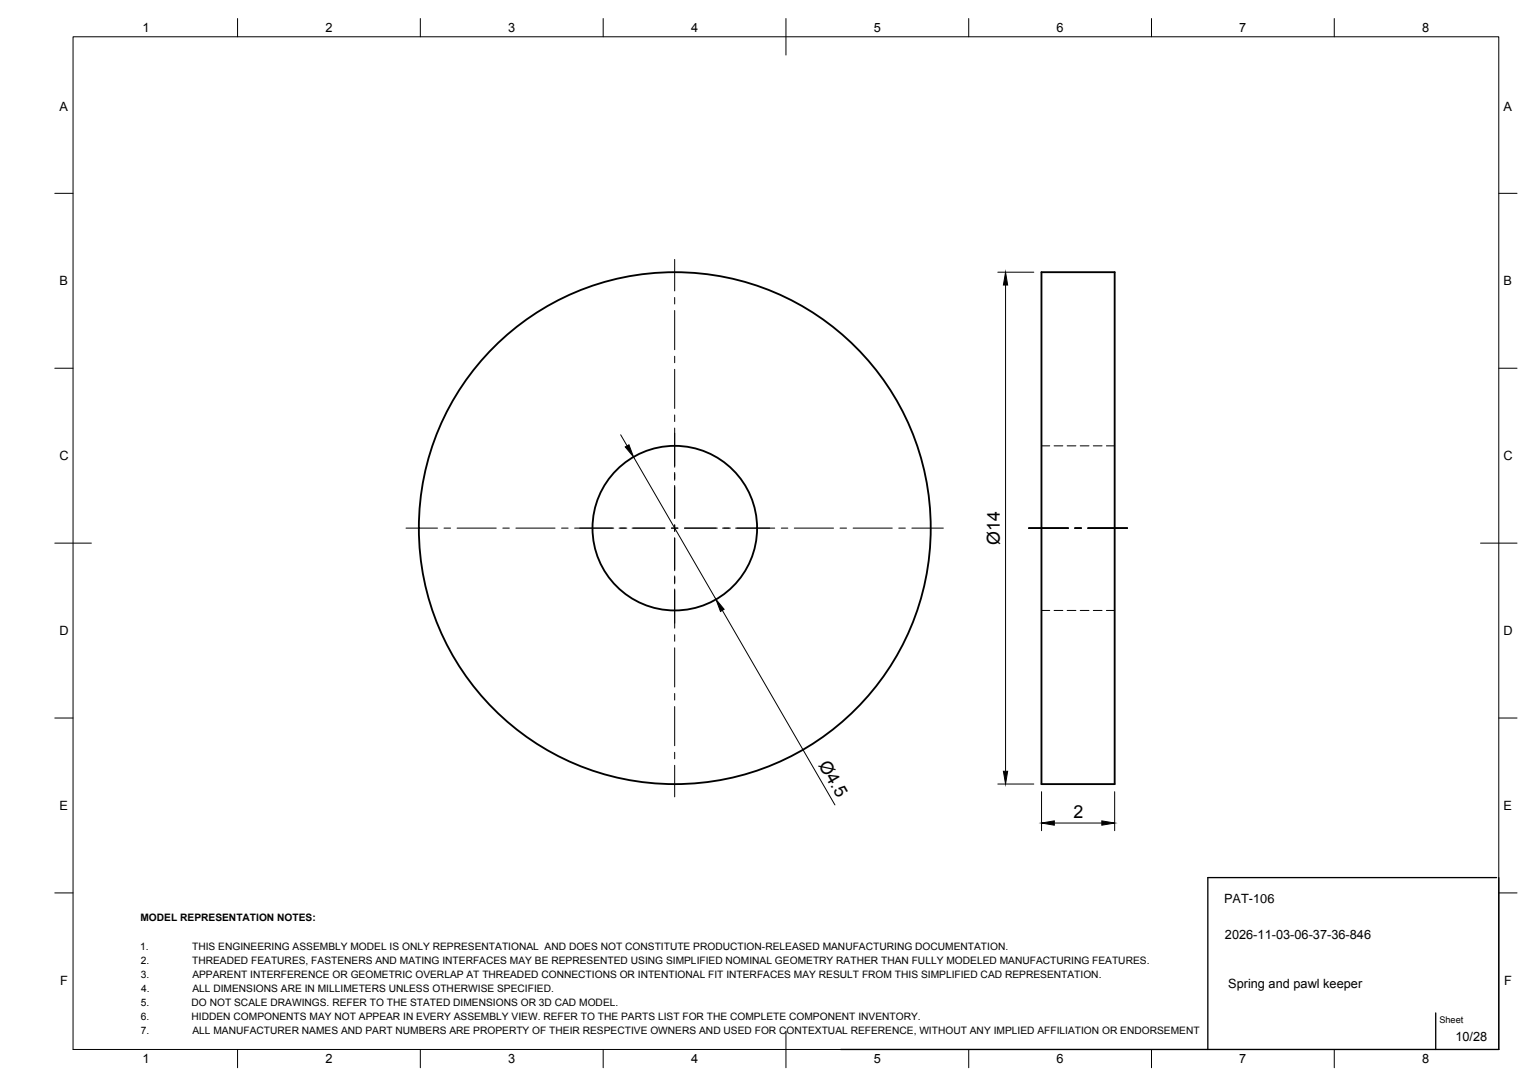
ISO-10303-21;
HEADER;
/* Generated by software containing ST-Developer
 * from STEP Tools, Inc. (www.steptools.com) 
 */

FILE_DESCRIPTION(
/* description */ ('Torsion-spring ratchet demonstrator'),
/* implementation_level */ '2;1');

FILE_NAME(
/* name */ 'Spring and pawl keeper.step',
/* time_stamp */ '2026-10-29T17:29:17-07:00',
/* author */ (''),
/* organization */ (''),
/* preprocessor_version */ 'ST-DEVELOPER v20.2',
/* originating_system */ 'Autodesk Translation Framework v15.17.0.0',
/* authorisation */ '');

FILE_SCHEMA (('AUTOMOTIVE_DESIGN { 1 0 10303 214 3 1 1 }'));
ENDSEC;

DATA;
#10=MECHANICAL_DESIGN_GEOMETRIC_PRESENTATION_REPRESENTATION('',(#288),#11258);
#240=SHAPE_REPRESENTATION_RELATIONSHIP('SRR','None',#11366,#264);
#264=ADVANCED_BREP_SHAPE_REPRESENTATION('',(#320),#11236);
#288=STYLED_ITEM('',(#11584),#320);
#320=MANIFOLD_SOLID_BREP('Body1',#5159);
#373=FACE_BOUND('',#1000,.T.);
#374=FACE_BOUND('',#1002,.T.);
#459=PLANE('',#5546);
#460=PLANE('',#5547);
#664=FACE_OUTER_BOUND('',#997,.T.);
#665=FACE_OUTER_BOUND('',#998,.T.);
#666=FACE_OUTER_BOUND('',#999,.T.);
#667=FACE_OUTER_BOUND('',#1001,.T.);
#997=EDGE_LOOP('',(#3604,#3605,#3606,#3607));
#998=EDGE_LOOP('',(#3608,#3609,#3610,#3611));
#999=EDGE_LOOP('',(#3612));
#1000=EDGE_LOOP('',(#3613));
#1001=EDGE_LOOP('',(#3614));
#1002=EDGE_LOOP('',(#3615));
#1368=LINE('',#7863,#1751);
#1369=LINE('',#7869,#1752);
#1751=VECTOR('',#6287,0.225);
#1752=VECTOR('',#6294,0.7);
#2129=CIRCLE('',#5541,0.225);
#2130=CIRCLE('',#5542,0.225);
#2131=CIRCLE('',#5544,0.7);
#2132=CIRCLE('',#5545,0.7);
#2389=VERTEX_POINT('',#7860);
#2390=VERTEX_POINT('',#7862);
#2391=VERTEX_POINT('',#7866);
#2392=VERTEX_POINT('',#7868);
#2862=EDGE_CURVE('',#2389,#2389,#2129,.T.);
#2863=EDGE_CURVE('',#2389,#2390,#1368,.T.);
#2864=EDGE_CURVE('',#2390,#2390,#2130,.T.);
#2865=EDGE_CURVE('',#2391,#2391,#2131,.T.);
#2866=EDGE_CURVE('',#2391,#2392,#1369,.T.);
#2867=EDGE_CURVE('',#2392,#2392,#2132,.T.);
#3604=ORIENTED_EDGE('',*,*,#2862,.F.);
#3605=ORIENTED_EDGE('',*,*,#2863,.T.);
#3606=ORIENTED_EDGE('',*,*,#2864,.T.);
#3607=ORIENTED_EDGE('',*,*,#2863,.F.);
#3608=ORIENTED_EDGE('',*,*,#2865,.F.);
#3609=ORIENTED_EDGE('',*,*,#2866,.T.);
#3610=ORIENTED_EDGE('',*,*,#2867,.T.);
#3611=ORIENTED_EDGE('',*,*,#2866,.F.);
#3612=ORIENTED_EDGE('',*,*,#2865,.T.);
#3613=ORIENTED_EDGE('',*,*,#2862,.T.);
#3614=ORIENTED_EDGE('',*,*,#2867,.F.);
#3615=ORIENTED_EDGE('',*,*,#2864,.F.);
#4783=CYLINDRICAL_SURFACE('',#5540,0.225);
#4784=CYLINDRICAL_SURFACE('',#5543,0.7);
#4890=ADVANCED_FACE('',(#664),#4783,.F.);
#4891=ADVANCED_FACE('',(#665),#4784,.T.);
#4892=ADVANCED_FACE('',(#666,#373),#459,.T.);
#4893=ADVANCED_FACE('',(#667,#374),#460,.F.);
#5159=CLOSED_SHELL('',(#4890,#4891,#4892,#4893));
#5539=AXIS2_PLACEMENT_3D('',#7858,#6281,#6282);
#5540=AXIS2_PLACEMENT_3D('',#7859,#6283,#6284);
#5541=AXIS2_PLACEMENT_3D('',#7861,#6285,#6286);
#5542=AXIS2_PLACEMENT_3D('',#7864,#6288,#6289);
#5543=AXIS2_PLACEMENT_3D('',#7865,#6290,#6291);
#5544=AXIS2_PLACEMENT_3D('',#7867,#6292,#6293);
#5545=AXIS2_PLACEMENT_3D('',#7870,#6295,#6296);
#5546=AXIS2_PLACEMENT_3D('',#7871,#6297,#6298);
#5547=AXIS2_PLACEMENT_3D('',#7872,#6299,#6300);
#6281=DIRECTION('axis',(0.,0.,1.));
#6282=DIRECTION('refdir',(1.,0.,0.));
#6283=DIRECTION('center_axis',(0.,0.,1.));
#6284=DIRECTION('ref_axis',(1.,0.,0.));
#6285=DIRECTION('center_axis',(0.,0.,-1.));
#6286=DIRECTION('ref_axis',(1.,0.,0.));
#6287=DIRECTION('',(0.,0.,-1.));
#6288=DIRECTION('center_axis',(0.,0.,-1.));
#6289=DIRECTION('ref_axis',(1.,0.,0.));
#6290=DIRECTION('center_axis',(0.,0.,1.));
#6291=DIRECTION('ref_axis',(1.,0.,0.));
#6292=DIRECTION('center_axis',(0.,0.,1.));
#6293=DIRECTION('ref_axis',(1.,0.,0.));
#6294=DIRECTION('',(0.,0.,-1.));
#6295=DIRECTION('center_axis',(0.,0.,1.));
#6296=DIRECTION('ref_axis',(1.,0.,0.));
#6297=DIRECTION('center_axis',(0.,0.,1.));
#6298=DIRECTION('ref_axis',(1.,0.,0.));
#6299=DIRECTION('center_axis',(0.,0.,1.));
#6300=DIRECTION('ref_axis',(1.,0.,0.));
#7858=CARTESIAN_POINT('',(0.,0.,0.));
#7859=CARTESIAN_POINT('Origin',(6.5,-3.47,6.64));
#7860=CARTESIAN_POINT('',(6.275,-3.47,6.84));
#7861=CARTESIAN_POINT('Origin',(6.5,-3.47,6.84));
#7862=CARTESIAN_POINT('',(6.275,-3.47,6.64));
#7863=CARTESIAN_POINT('',(6.275,-3.47,6.64));
#7864=CARTESIAN_POINT('Origin',(6.5,-3.47,6.64));
#7865=CARTESIAN_POINT('Origin',(6.5,-3.47,6.64));
#7866=CARTESIAN_POINT('',(5.8,-3.47,6.84));
#7867=CARTESIAN_POINT('Origin',(6.5,-3.47,6.84));
#7868=CARTESIAN_POINT('',(5.8,-3.47,6.64));
#7869=CARTESIAN_POINT('',(5.8,-3.47,6.64));
#7870=CARTESIAN_POINT('Origin',(6.5,-3.47,6.64));
#7871=CARTESIAN_POINT('Origin',(6.5,-3.47,6.84));
#7872=CARTESIAN_POINT('Origin',(6.5,-3.47,6.64));
#11206=UNCERTAINTY_MEASURE_WITH_UNIT(LENGTH_MEASURE(0.001),#11259,
'DISTANCE_ACCURACY_VALUE',
'Maximum model space distance between geometric entities at asserted c
onnectivities');
#11228=UNCERTAINTY_MEASURE_WITH_UNIT(LENGTH_MEASURE(0.001),#11259,
'DISTANCE_ACCURACY_VALUE',
'Maximum model space distance between geometric entities at asserted c
onnectivities');
#11236=(
GEOMETRIC_REPRESENTATION_CONTEXT(3)
GLOBAL_UNCERTAINTY_ASSIGNED_CONTEXT((#11206))
GLOBAL_UNIT_ASSIGNED_CONTEXT((#11259,#11261,#11262))
REPRESENTATION_CONTEXT('','3D')
);
#11258=(
GEOMETRIC_REPRESENTATION_CONTEXT(3)
GLOBAL_UNCERTAINTY_ASSIGNED_CONTEXT((#11228))
GLOBAL_UNIT_ASSIGNED_CONTEXT((#11259,#11261,#11262))
REPRESENTATION_CONTEXT('','3D')
);
#11259=(
LENGTH_UNIT()
NAMED_UNIT(*)
SI_UNIT(.CENTI.,.METRE.)
);
#11261=(
NAMED_UNIT(*)
PLANE_ANGLE_UNIT()
SI_UNIT($,.RADIAN.)
);
#11262=(
NAMED_UNIT(*)
SI_UNIT($,.STERADIAN.)
SOLID_ANGLE_UNIT()
);
#11270=SHAPE_DEFINITION_REPRESENTATION(#11299,#11366);
#11299=PRODUCT_DEFINITION_SHAPE('',$,#11396);
#11366=SHAPE_REPRESENTATION('',(#5539),#11236);
#11388=PRODUCT_DEFINITION_CONTEXT('part definition',#11477,'design');
#11396=PRODUCT_DEFINITION('Spring and pawl keeper',
'Spring and pawl keeper',#11425,#11388);
#11425=PRODUCT_DEFINITION_FORMATION('',$,#11486);
#11477=APPLICATION_CONTEXT(
'Core Data for Automotive Mechanical Design Process');
#11478=PRODUCT_CONTEXT('part definition',#11477,'mechanical');
#11486=PRODUCT('Spring and pawl keeper','Spring and pawl keeper',
'Spring and pawl keeper',(#11478));
#11578=COLOUR_RGB('Grey',0.48,0.52,0.57);
#11579=FILL_AREA_STYLE_COLOUR('',#11578);
#11580=FILL_AREA_STYLE('',(#11579));
#11581=SURFACE_STYLE_FILL_AREA(#11580);
#11582=SURFACE_SIDE_STYLE('',(#11581));
#11583=SURFACE_STYLE_USAGE(.BOTH.,#11582);
#11584=PRESENTATION_STYLE_ASSIGNMENT((#11583));
ENDSEC;
END-ISO-10303-21;
